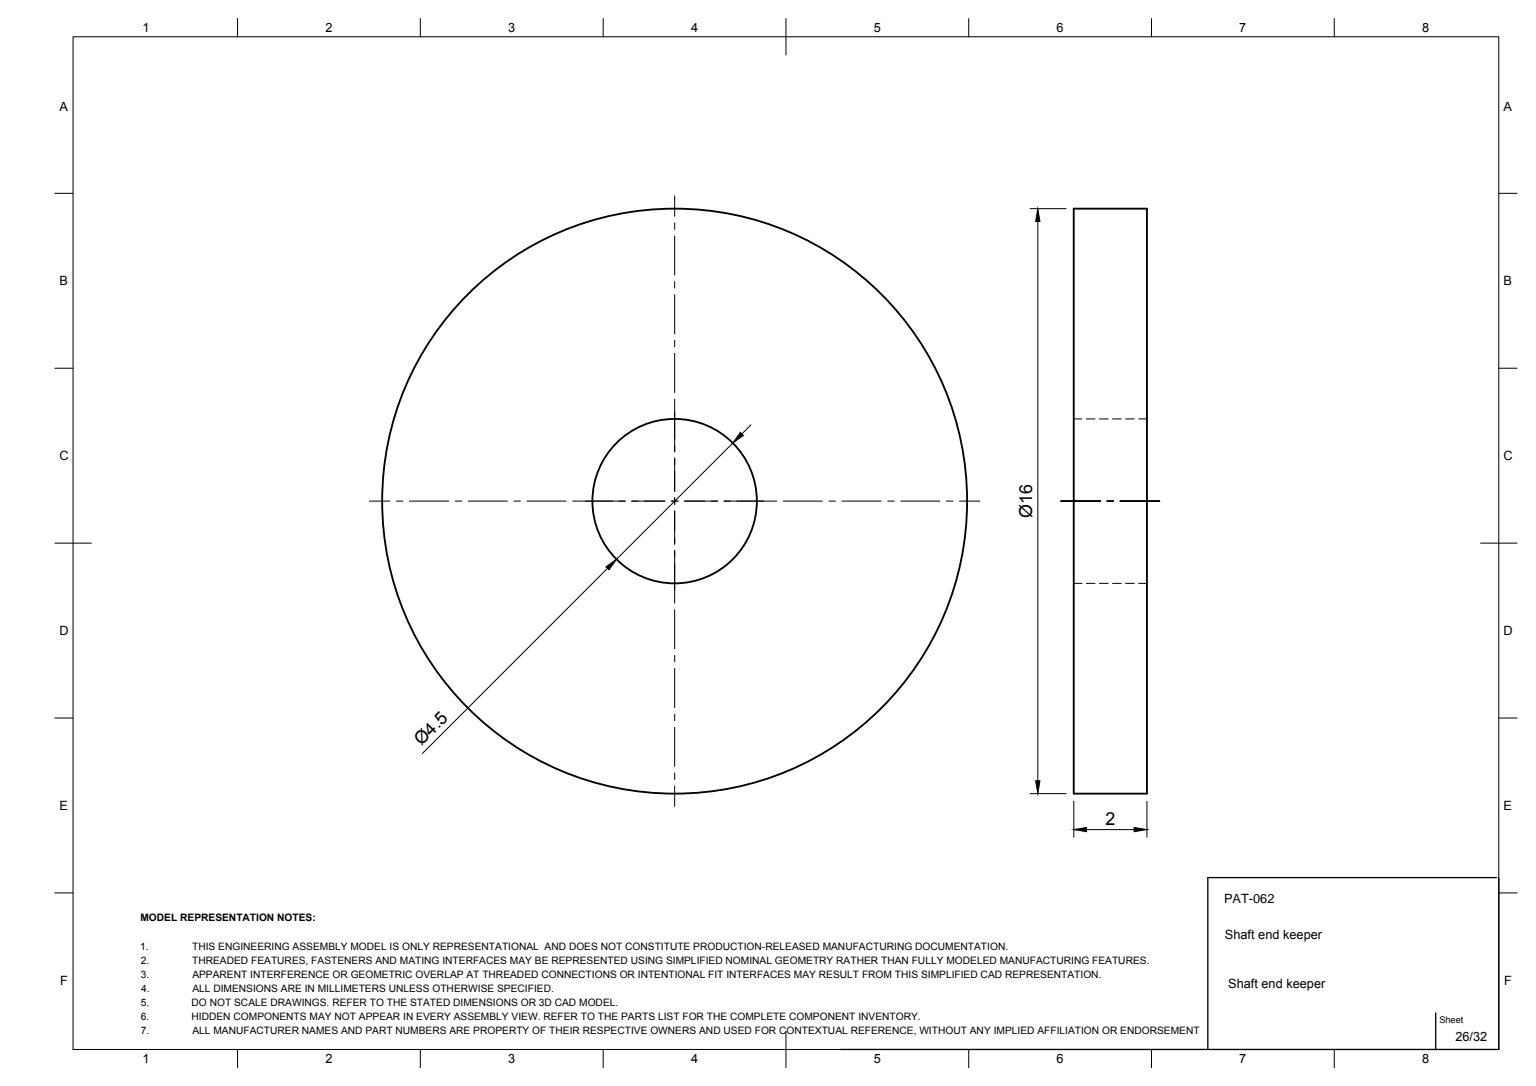
ISO-10303-21;
HEADER;
/* Generated by software containing ST-Developer
 * from STEP Tools, Inc. (www.steptools.com) 
 */

FILE_DESCRIPTION(
/* description */ ('Jaw-coupled motor to shaft test stand'),
/* implementation_level */ '2;1');

FILE_NAME(
/* name */ 'Shaft end keeper.step',
/* time_stamp */ '2026-10-27T10:46:06-07:00',
/* author */ (''),
/* organization */ (''),
/* preprocessor_version */ 'ST-DEVELOPER v20.2',
/* originating_system */ 'Autodesk Translation Framework v15.17.0.0',
/* authorisation */ '');

FILE_SCHEMA (('AUTOMOTIVE_DESIGN { 1 0 10303 214 3 1 1 }'));
ENDSEC;

DATA;
#10=MECHANICAL_DESIGN_GEOMETRIC_PRESENTATION_REPRESENTATION('',(#365),#19361);
#300=SHAPE_REPRESENTATION_RELATIONSHIP('SRR','None',#19516,#332);
#332=ADVANCED_BREP_SHAPE_REPRESENTATION('',(#396),#19352);
#365=STYLED_ITEM('',(#19746),#396);
#396=MANIFOLD_SOLID_BREP('Body1',#11011);
#503=FACE_BOUND('',#1994,.T.);
#504=FACE_BOUND('',#1996,.T.);
#683=PLANE('',#11844);
#684=PLANE('',#11845);
#1271=FACE_OUTER_BOUND('',#1991,.T.);
#1272=FACE_OUTER_BOUND('',#1992,.T.);
#1273=FACE_OUTER_BOUND('',#1993,.T.);
#1274=FACE_OUTER_BOUND('',#1995,.T.);
#1991=EDGE_LOOP('',(#8412,#8413,#8414,#8415));
#1992=EDGE_LOOP('',(#8416,#8417,#8418,#8419));
#1993=EDGE_LOOP('',(#8420));
#1994=EDGE_LOOP('',(#8421));
#1995=EDGE_LOOP('',(#8422));
#1996=EDGE_LOOP('',(#8423));
#2708=LINE('',#17247,#3861);
#2709=LINE('',#17253,#3862);
#3861=VECTOR('',#13607,0.225);
#3862=VECTOR('',#13614,0.8);
#4841=CIRCLE('',#11839,0.225);
#4842=CIRCLE('',#11840,0.225);
#4843=CIRCLE('',#11842,0.8);
#4844=CIRCLE('',#11843,0.8);
#5305=VERTEX_POINT('',#17244);
#5306=VERTEX_POINT('',#17246);
#5307=VERTEX_POINT('',#17250);
#5308=VERTEX_POINT('',#17252);
#6417=EDGE_CURVE('',#5305,#5305,#4841,.T.);
#6418=EDGE_CURVE('',#5305,#5306,#2708,.T.);
#6419=EDGE_CURVE('',#5306,#5306,#4842,.T.);
#6420=EDGE_CURVE('',#5307,#5307,#4843,.T.);
#6421=EDGE_CURVE('',#5307,#5308,#2709,.T.);
#6422=EDGE_CURVE('',#5308,#5308,#4844,.T.);
#8412=ORIENTED_EDGE('',*,*,#6417,.F.);
#8413=ORIENTED_EDGE('',*,*,#6418,.T.);
#8414=ORIENTED_EDGE('',*,*,#6419,.T.);
#8415=ORIENTED_EDGE('',*,*,#6418,.F.);
#8416=ORIENTED_EDGE('',*,*,#6420,.F.);
#8417=ORIENTED_EDGE('',*,*,#6421,.T.);
#8418=ORIENTED_EDGE('',*,*,#6422,.T.);
#8419=ORIENTED_EDGE('',*,*,#6421,.F.);
#8420=ORIENTED_EDGE('',*,*,#6420,.T.);
#8421=ORIENTED_EDGE('',*,*,#6417,.T.);
#8422=ORIENTED_EDGE('',*,*,#6422,.F.);
#8423=ORIENTED_EDGE('',*,*,#6419,.F.);
#10344=CYLINDRICAL_SURFACE('',#11838,0.225);
#10345=CYLINDRICAL_SURFACE('',#11841,0.8);
#10613=ADVANCED_FACE('',(#1271),#10344,.F.);
#10614=ADVANCED_FACE('',(#1272),#10345,.T.);
#10615=ADVANCED_FACE('',(#1273,#503),#683,.T.);
#10616=ADVANCED_FACE('',(#1274,#504),#684,.F.);
#11011=CLOSED_SHELL('',(#10613,#10614,#10615,#10616));
#11837=AXIS2_PLACEMENT_3D('',#17242,#13601,#13602);
#11838=AXIS2_PLACEMENT_3D('',#17243,#13603,#13604);
#11839=AXIS2_PLACEMENT_3D('',#17245,#13605,#13606);
#11840=AXIS2_PLACEMENT_3D('',#17248,#13608,#13609);
#11841=AXIS2_PLACEMENT_3D('',#17249,#13610,#13611);
#11842=AXIS2_PLACEMENT_3D('',#17251,#13612,#13613);
#11843=AXIS2_PLACEMENT_3D('',#17254,#13615,#13616);
#11844=AXIS2_PLACEMENT_3D('',#17255,#13617,#13618);
#11845=AXIS2_PLACEMENT_3D('',#17256,#13619,#13620);
#13601=DIRECTION('axis',(0.,0.,1.));
#13602=DIRECTION('refdir',(1.,0.,0.));
#13603=DIRECTION('center_axis',(0.,1.,0.));
#13604=DIRECTION('ref_axis',(1.,0.,0.));
#13605=DIRECTION('center_axis',(0.,-1.,0.));
#13606=DIRECTION('ref_axis',(1.,0.,0.));
#13607=DIRECTION('',(0.,-1.,0.));
#13608=DIRECTION('center_axis',(0.,-1.,0.));
#13609=DIRECTION('ref_axis',(1.,0.,0.));
#13610=DIRECTION('center_axis',(0.,1.,0.));
#13611=DIRECTION('ref_axis',(1.,0.,0.));
#13612=DIRECTION('center_axis',(0.,1.,0.));
#13613=DIRECTION('ref_axis',(1.,0.,0.));
#13614=DIRECTION('',(0.,-1.,0.));
#13615=DIRECTION('center_axis',(0.,1.,0.));
#13616=DIRECTION('ref_axis',(1.,0.,0.));
#13617=DIRECTION('center_axis',(0.,1.,0.));
#13618=DIRECTION('ref_axis',(1.,0.,0.));
#13619=DIRECTION('center_axis',(0.,1.,0.));
#13620=DIRECTION('ref_axis',(1.,0.,0.));
#17242=CARTESIAN_POINT('',(0.,0.,0.));
#17243=CARTESIAN_POINT('Origin',(0.,22.,4.22));
#17244=CARTESIAN_POINT('',(-0.225,22.2,4.22));
#17245=CARTESIAN_POINT('Origin',(0.,22.2,4.22));
#17246=CARTESIAN_POINT('',(-0.225,22.,4.22));
#17247=CARTESIAN_POINT('',(-0.225,22.,4.22));
#17248=CARTESIAN_POINT('Origin',(0.,22.,4.22));
#17249=CARTESIAN_POINT('Origin',(0.,22.,4.22));
#17250=CARTESIAN_POINT('',(-0.8,22.2,4.22));
#17251=CARTESIAN_POINT('Origin',(0.,22.2,4.22));
#17252=CARTESIAN_POINT('',(-0.8,22.,4.22));
#17253=CARTESIAN_POINT('',(-0.8,22.,4.22));
#17254=CARTESIAN_POINT('Origin',(0.,22.,4.22));
#17255=CARTESIAN_POINT('Origin',(0.,22.2,4.22));
#17256=CARTESIAN_POINT('Origin',(0.,22.,4.22));
#19314=UNCERTAINTY_MEASURE_WITH_UNIT(LENGTH_MEASURE(0.001),#19362,
'DISTANCE_ACCURACY_VALUE',
'Maximum model space distance between geometric entities at asserted c
onnectivities');
#19323=UNCERTAINTY_MEASURE_WITH_UNIT(LENGTH_MEASURE(0.001),#19362,
'DISTANCE_ACCURACY_VALUE',
'Maximum model space distance between geometric entities at asserted c
onnectivities');
#19352=(
GEOMETRIC_REPRESENTATION_CONTEXT(3)
GLOBAL_UNCERTAINTY_ASSIGNED_CONTEXT((#19314))
GLOBAL_UNIT_ASSIGNED_CONTEXT((#19362,#19364,#19365))
REPRESENTATION_CONTEXT('','3D')
);
#19361=(
GEOMETRIC_REPRESENTATION_CONTEXT(3)
GLOBAL_UNCERTAINTY_ASSIGNED_CONTEXT((#19323))
GLOBAL_UNIT_ASSIGNED_CONTEXT((#19362,#19364,#19365))
REPRESENTATION_CONTEXT('','3D')
);
#19362=(
LENGTH_UNIT()
NAMED_UNIT(*)
SI_UNIT(.CENTI.,.METRE.)
);
#19364=(
NAMED_UNIT(*)
PLANE_ANGLE_UNIT()
SI_UNIT($,.RADIAN.)
);
#19365=(
NAMED_UNIT(*)
SI_UNIT($,.STERADIAN.)
SOLID_ANGLE_UNIT()
);
#19394=SHAPE_DEFINITION_REPRESENTATION(#19458,#19516);
#19458=PRODUCT_DEFINITION_SHAPE('',$,#19554);
#19516=SHAPE_REPRESENTATION('',(#11837),#19352);
#19525=PRODUCT_DEFINITION_CONTEXT('part definition',#19638,'design');
#19554=PRODUCT_DEFINITION('Shaft end keeper','Shaft end keeper',#19591,
#19525);
#19591=PRODUCT_DEFINITION_FORMATION('',$,#19668);
#19638=APPLICATION_CONTEXT(
'Core Data for Automotive Mechanical Design Process');
#19639=PRODUCT_CONTEXT('part definition',#19638,'mechanical');
#19668=PRODUCT('Shaft end keeper','Shaft end keeper','Shaft end keeper',
(#19639));
#19740=COLOUR_RGB('Grey',0.48,0.52,0.57);
#19741=FILL_AREA_STYLE_COLOUR('',#19740);
#19742=FILL_AREA_STYLE('',(#19741));
#19743=SURFACE_STYLE_FILL_AREA(#19742);
#19744=SURFACE_SIDE_STYLE('',(#19743));
#19745=SURFACE_STYLE_USAGE(.BOTH.,#19744);
#19746=PRESENTATION_STYLE_ASSIGNMENT((#19745));
ENDSEC;
END-ISO-10303-21;
